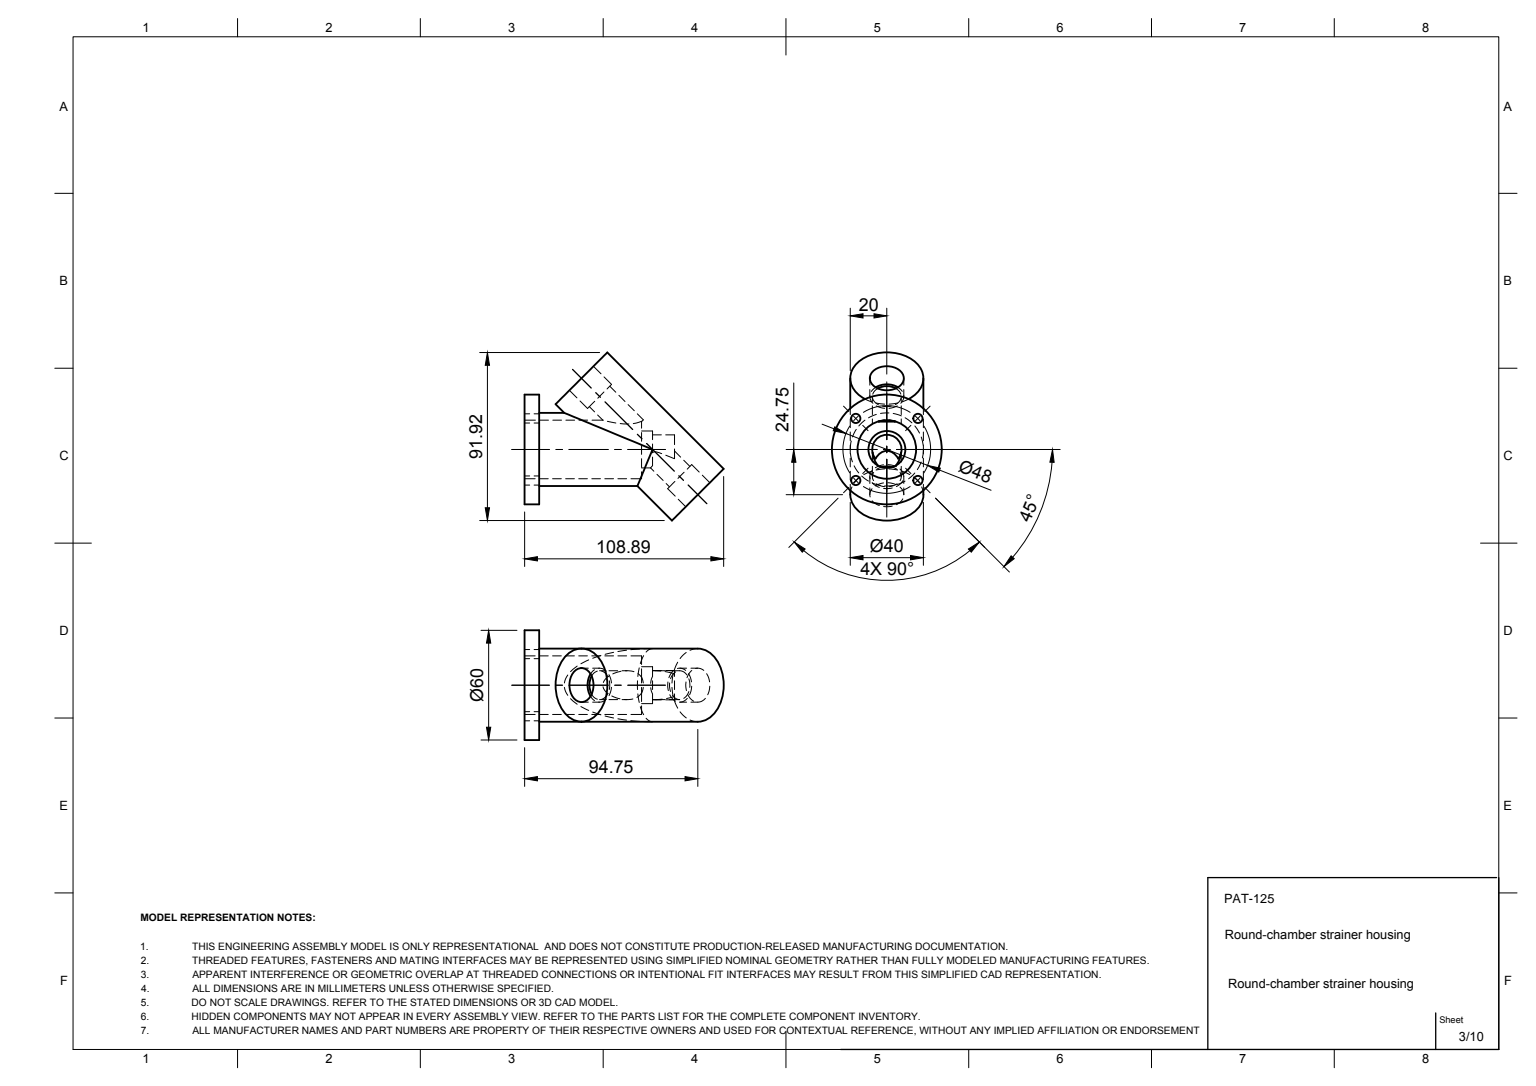
ISO-10303-21;
HEADER;
/* Generated by software containing ST-Developer
 * from STEP Tools, Inc. (www.steptools.com) 
 */

FILE_DESCRIPTION(
/* description */ ('Y-strainer with drain'),
/* implementation_level */ '2;1');

FILE_NAME(
/* name */ 'Round-chamber strainer housing.step',
/* time_stamp */ '2026-10-28T00:41:55-07:00',
/* author */ (''),
/* organization */ (''),
/* preprocessor_version */ 'ST-DEVELOPER v20.2',
/* originating_system */ 'Autodesk Translation Framework v15.17.0.0',
/* authorisation */ '');

FILE_SCHEMA (('AUTOMOTIVE_DESIGN { 1 0 10303 214 3 1 1 }'));
ENDSEC;

DATA;
#10=MECHANICAL_DESIGN_GEOMETRIC_PRESENTATION_REPRESENTATION('',(#93),#8864);
#75=SHAPE_REPRESENTATION_RELATIONSHIP('SRR','None',#8907,#84);
#84=ADVANCED_BREP_SHAPE_REPRESENTATION('',(#102),#8855);
#93=STYLED_ITEM('',(#9012),#102);
#102=MANIFOLD_SOLID_BREP('Body1',#3383);
#110=B_SPLINE_CURVE_WITH_KNOTS('',3,(#4530,#4531,#4532,#4533,#4534,#4535,
#4536,#4537,#4538,#4539,#4540,#4541,#4542,#4543,#4544,#4545,#4546,#4547,
#4548,#4549),.UNSPECIFIED.,.F.,.F.,(4,2,2,2,2,2,2,2,2,4),(-4.14934014091753,
-3.99654801890952,-3.81097439305959,-3.62540076720966,-3.2542535155098,
-2.75110698726675,-2.2479604590237,-1.9375436083893,-1.7823351830721,-1.6271267577549),
 .UNSPECIFIED.);
#111=B_SPLINE_CURVE_WITH_KNOTS('',3,(#4550,#4551,#4552,#4553,#4554,#4555,
#4556,#4557,#4558,#4559,#4560,#4561,#4562,#4563,#4564,#4565,#4566,#4567,
#4568,#4569,#4570),.UNSPECIFIED.,.F.,.F.,(4,2,2,2,2,3,2,2,2,4),(-1.6271267577549,
-1.4719183324377,-1.3167099071205,-1.00629305648611,-0.503146528243052,
0.,0.371147251699857,0.556720877549785,0.742294503399713,0.895086625004965),
 .UNSPECIFIED.);
#112=B_SPLINE_CURVE_WITH_KNOTS('',3,(#4581,#4582,#4583,#4584,#4585,#4586,
#4587,#4588,#4589,#4590),.UNSPECIFIED.,.F.,.F.,(4,2,2,2,4),(1.74412062919654,
1.93171537626907,2.23482107464905,2.53792677302904,2.72552152010157),
 .UNSPECIFIED.);
#113=B_SPLINE_CURVE_WITH_KNOTS('',3,(#4608,#4609,#4610,#4611,#4612,#4613,
#4614,#4615,#4616,#4617,#4618,#4619,#4620,#4621,#4622,#4623,#4624,#4625,
#4626),.UNSPECIFIED.,.F.,.F.,(4,2,2,2,2,3,2,2,4),(-1.08793576529359,-1.02464359039736,
-0.589129183459348,-0.223538305364611,-0.111769152682306,0.,0.0571948520978316,
0.114389704195663,0.138769598257235),.UNSPECIFIED.);
#114=B_SPLINE_CURVE_WITH_KNOTS('',3,(#4628,#4629,#4630,#4631,#4632,#4633,
#4634,#4635,#4636,#4637,#4638,#4639,#4640,#4641,#4642,#4643,#4644,#4645),
 .UNSPECIFIED.,.F.,.F.,(4,2,2,2,2,2,2,2,4),(2.32433792360818,2.34871781766975,
2.40591266976758,2.46310752186541,2.57487667454772,2.68664582723002,3.05223670532476,
3.48775111226277,3.551043287159),.UNSPECIFIED.);
#319=FACE_BOUND('',#677,.T.);
#320=FACE_BOUND('',#687,.T.);
#321=FACE_BOUND('',#690,.T.);
#322=FACE_BOUND('',#693,.T.);
#323=FACE_BOUND('',#694,.T.);
#324=FACE_BOUND('',#695,.T.);
#325=FACE_BOUND('',#696,.T.);
#326=FACE_BOUND('',#697,.T.);
#327=FACE_BOUND('',#701,.T.);
#328=FACE_BOUND('',#702,.T.);
#329=FACE_BOUND('',#703,.T.);
#330=FACE_BOUND('',#704,.T.);
#331=FACE_BOUND('',#705,.T.);
#332=FACE_BOUND('',#707,.T.);
#333=FACE_BOUND('',#709,.T.);
#334=FACE_BOUND('',#711,.T.);
#456=ELLIPSE('',#3509,1.11722871427475,0.79);
#457=ELLIPSE('',#3511,1.11722871427475,0.79);
#458=ELLIPSE('',#3522,1.11722871427475,0.79);
#459=ELLIPSE('',#3524,1.11722871427475,0.79);
#460=ELLIPSE('',#3527,1.11722871427475,0.79);
#461=ELLIPSE('',#3528,1.11722871427475,0.79);
#462=ELLIPSE('',#3548,5.22625185950551,2.);
#463=ELLIPSE('',#3549,2.16478440058479,2.);
#464=ELLIPSE('',#3550,5.22625185950551,2.);
#465=PLANE('',#3508);
#466=PLANE('',#3515);
#467=PLANE('',#3521);
#468=PLANE('',#3529);
#469=PLANE('',#3535);
#470=PLANE('',#3540);
#471=PLANE('',#3542);
#472=PLANE('',#3551);
#473=PLANE('',#3555);
#474=PLANE('',#3556);
#520=FACE_OUTER_BOUND('',#672,.T.);
#521=FACE_OUTER_BOUND('',#673,.T.);
#522=FACE_OUTER_BOUND('',#674,.T.);
#523=FACE_OUTER_BOUND('',#675,.T.);
#524=FACE_OUTER_BOUND('',#676,.T.);
#525=FACE_OUTER_BOUND('',#678,.T.);
#526=FACE_OUTER_BOUND('',#679,.T.);
#527=FACE_OUTER_BOUND('',#680,.T.);
#528=FACE_OUTER_BOUND('',#681,.T.);
#529=FACE_OUTER_BOUND('',#682,.T.);
#530=FACE_OUTER_BOUND('',#683,.T.);
#531=FACE_OUTER_BOUND('',#684,.T.);
#532=FACE_OUTER_BOUND('',#685,.T.);
#533=FACE_OUTER_BOUND('',#686,.T.);
#534=FACE_OUTER_BOUND('',#688,.T.);
#535=FACE_OUTER_BOUND('',#689,.T.);
#536=FACE_OUTER_BOUND('',#691,.T.);
#537=FACE_OUTER_BOUND('',#692,.T.);
#538=FACE_OUTER_BOUND('',#698,.T.);
#539=FACE_OUTER_BOUND('',#699,.T.);
#540=FACE_OUTER_BOUND('',#700,.T.);
#541=FACE_OUTER_BOUND('',#706,.T.);
#542=FACE_OUTER_BOUND('',#708,.T.);
#543=FACE_OUTER_BOUND('',#710,.T.);
#672=EDGE_LOOP('',(#2194,#2195,#2196,#2197));
#673=EDGE_LOOP('',(#2198,#2199,#2200,#2201));
#674=EDGE_LOOP('',(#2202,#2203,#2204,#2205));
#675=EDGE_LOOP('',(#2206,#2207,#2208,#2209));
#676=EDGE_LOOP('',(#2210,#2211,#2212,#2213));
#677=EDGE_LOOP('',(#2214));
#678=EDGE_LOOP('',(#2215,#2216,#2217,#2218,#2219,#2220));
#679=EDGE_LOOP('',(#2221,#2222,#2223));
#680=EDGE_LOOP('',(#2224,#2225,#2226,#2227,#2228,#2229));
#681=EDGE_LOOP('',(#2230,#2231,#2232,#2233,#2234));
#682=EDGE_LOOP('',(#2235,#2236,#2237,#2238,#2239,#2240,#2241,#2242,#2243,
#2244));
#683=EDGE_LOOP('',(#2245,#2246,#2247));
#684=EDGE_LOOP('',(#2248,#2249,#2250,#2251));
#685=EDGE_LOOP('',(#2252,#2253,#2254,#2255));
#686=EDGE_LOOP('',(#2256));
#687=EDGE_LOOP('',(#2257));
#688=EDGE_LOOP('',(#2258,#2259,#2260,#2261));
#689=EDGE_LOOP('',(#2262));
#690=EDGE_LOOP('',(#2263));
#691=EDGE_LOOP('',(#2264,#2265,#2266,#2267,#2268,#2269,#2270,#2271,#2272));
#692=EDGE_LOOP('',(#2273));
#693=EDGE_LOOP('',(#2274));
#694=EDGE_LOOP('',(#2275));
#695=EDGE_LOOP('',(#2276));
#696=EDGE_LOOP('',(#2277));
#697=EDGE_LOOP('',(#2278));
#698=EDGE_LOOP('',(#2279,#2280,#2281,#2282));
#699=EDGE_LOOP('',(#2283,#2284,#2285,#2286,#2287,#2288));
#700=EDGE_LOOP('',(#2289));
#701=EDGE_LOOP('',(#2290));
#702=EDGE_LOOP('',(#2291));
#703=EDGE_LOOP('',(#2292));
#704=EDGE_LOOP('',(#2293));
#705=EDGE_LOOP('',(#2294));
#706=EDGE_LOOP('',(#2295,#2296,#2297,#2298));
#707=EDGE_LOOP('',(#2299,#2300,#2301));
#708=EDGE_LOOP('',(#2302));
#709=EDGE_LOOP('',(#2303));
#710=EDGE_LOOP('',(#2304));
#711=EDGE_LOOP('',(#2305));
#961=LINE('',#4497,#1124);
#962=LINE('',#4503,#1125);
#963=LINE('',#4509,#1126);
#964=LINE('',#4515,#1127);
#965=LINE('',#4525,#1128);
#966=LINE('',#4572,#1129);
#967=LINE('',#4593,#1130);
#968=LINE('',#4605,#1131);
#969=LINE('',#4654,#1132);
#970=LINE('',#4663,#1133);
#971=LINE('',#4667,#1134);
#972=LINE('',#4676,#1135);
#973=LINE('',#4679,#1136);
#974=LINE('',#4690,#1137);
#1124=VECTOR('',#3781,0.25);
#1125=VECTOR('',#3788,0.25);
#1126=VECTOR('',#3795,0.25);
#1127=VECTOR('',#3802,0.25);
#1128=VECTOR('',#3813,1.);
#1129=VECTOR('',#3818,1.6);
#1130=VECTOR('',#3831,1.01);
#1131=VECTOR('',#3846,0.79);
#1132=VECTOR('',#3861,0.93);
#1133=VECTOR('',#3872,0.93);
#1134=VECTOR('',#3879,0.79);
#1135=VECTOR('',#3890,3.);
#1136=VECTOR('',#3893,2.);
#1137=VECTOR('',#3906,2.);
#1287=CIRCLE('',#3497,0.25);
#1288=CIRCLE('',#3498,0.25);
#1289=CIRCLE('',#3500,0.25);
#1290=CIRCLE('',#3501,0.25);
#1291=CIRCLE('',#3503,0.25);
#1292=CIRCLE('',#3504,0.25);
#1293=CIRCLE('',#3506,0.25);
#1294=CIRCLE('',#3507,0.25);
#1295=CIRCLE('',#3510,1.6);
#1296=CIRCLE('',#3512,1.01);
#1297=CIRCLE('',#3514,1.6);
#1298=CIRCLE('',#3516,0.79);
#1299=CIRCLE('',#3517,0.79);
#1300=CIRCLE('',#3519,1.01);
#1301=CIRCLE('',#3520,1.01);
#1302=CIRCLE('',#3523,0.8);
#1303=CIRCLE('',#3526,0.79);
#1304=CIRCLE('',#3530,0.8);
#1305=CIRCLE('',#3533,0.93);
#1306=CIRCLE('',#3534,0.93);
#1307=CIRCLE('',#3536,0.79);
#1308=CIRCLE('',#3538,0.93);
#1309=CIRCLE('',#3539,0.93);
#1310=CIRCLE('',#3543,3.);
#1311=CIRCLE('',#3544,2.);
#1312=CIRCLE('',#3546,3.);
#1313=CIRCLE('',#3553,2.);
#1314=CIRCLE('',#3554,2.);
#1379=VERTEX_POINT('',#4494);
#1380=VERTEX_POINT('',#4496);
#1381=VERTEX_POINT('',#4500);
#1382=VERTEX_POINT('',#4502);
#1383=VERTEX_POINT('',#4506);
#1384=VERTEX_POINT('',#4508);
#1385=VERTEX_POINT('',#4512);
#1386=VERTEX_POINT('',#4514);
#1387=VERTEX_POINT('',#4518);
#1388=VERTEX_POINT('',#4519);
#1389=VERTEX_POINT('',#4521);
#1390=VERTEX_POINT('',#4523);
#1391=VERTEX_POINT('',#4526);
#1392=VERTEX_POINT('',#4529);
#1393=VERTEX_POINT('',#4571);
#1394=VERTEX_POINT('',#4575);
#1395=VERTEX_POINT('',#4579);
#1396=VERTEX_POINT('',#4580);
#1397=VERTEX_POINT('',#4591);
#1398=VERTEX_POINT('',#4596);
#1399=VERTEX_POINT('',#4598);
#1400=VERTEX_POINT('',#4602);
#1401=VERTEX_POINT('',#4604);
#1402=VERTEX_POINT('',#4606);
#1403=VERTEX_POINT('',#4627);
#1404=VERTEX_POINT('',#4651);
#1405=VERTEX_POINT('',#4653);
#1406=VERTEX_POINT('',#4657);
#1407=VERTEX_POINT('',#4660);
#1408=VERTEX_POINT('',#4662);
#1409=VERTEX_POINT('',#4669);
#1410=VERTEX_POINT('',#4671);
#1411=VERTEX_POINT('',#4674);
#1412=VERTEX_POINT('',#4678);
#1413=VERTEX_POINT('',#4680);
#1414=VERTEX_POINT('',#4682);
#1415=VERTEX_POINT('',#4687);
#1416=VERTEX_POINT('',#4689);
#1721=EDGE_CURVE('',#1379,#1379,#1287,.T.);
#1722=EDGE_CURVE('',#1379,#1380,#961,.T.);
#1723=EDGE_CURVE('',#1380,#1380,#1288,.T.);
#1724=EDGE_CURVE('',#1381,#1381,#1289,.T.);
#1725=EDGE_CURVE('',#1381,#1382,#962,.T.);
#1726=EDGE_CURVE('',#1382,#1382,#1290,.T.);
#1727=EDGE_CURVE('',#1383,#1383,#1291,.T.);
#1728=EDGE_CURVE('',#1383,#1384,#963,.T.);
#1729=EDGE_CURVE('',#1384,#1384,#1292,.T.);
#1730=EDGE_CURVE('',#1385,#1385,#1293,.T.);
#1731=EDGE_CURVE('',#1385,#1386,#964,.T.);
#1732=EDGE_CURVE('',#1386,#1386,#1294,.T.);
#1733=EDGE_CURVE('',#1387,#1388,#456,.T.);
#1734=EDGE_CURVE('',#1387,#1389,#1295,.T.);
#1735=EDGE_CURVE('',#1390,#1389,#457,.T.);
#1736=EDGE_CURVE('',#1388,#1390,#965,.T.);
#1737=EDGE_CURVE('',#1391,#1391,#1296,.T.);
#1738=EDGE_CURVE('',#1389,#1392,#110,.T.);
#1739=EDGE_CURVE('',#1392,#1387,#111,.T.);
#1740=EDGE_CURVE('',#1392,#1393,#966,.T.);
#1741=EDGE_CURVE('',#1393,#1393,#1297,.T.);
#1742=EDGE_CURVE('',#1390,#1394,#1298,.T.);
#1743=EDGE_CURVE('',#1394,#1388,#1299,.T.);
#1744=EDGE_CURVE('',#1395,#1396,#112,.T.);
#1745=EDGE_CURVE('',#1397,#1395,#1300,.T.);
#1746=EDGE_CURVE('',#1397,#1391,#967,.T.);
#1747=EDGE_CURVE('',#1396,#1397,#1301,.T.);
#1748=EDGE_CURVE('',#1398,#1395,#458,.T.);
#1749=EDGE_CURVE('',#1399,#1398,#1302,.T.);
#1750=EDGE_CURVE('',#1396,#1399,#459,.T.);
#1751=EDGE_CURVE('',#1400,#1400,#1303,.T.);
#1752=EDGE_CURVE('',#1400,#1401,#968,.T.);
#1753=EDGE_CURVE('',#1401,#1402,#460,.T.);
#1754=EDGE_CURVE('',#1402,#1398,#113,.T.);
#1755=EDGE_CURVE('',#1399,#1403,#114,.T.);
#1756=EDGE_CURVE('',#1403,#1401,#461,.T.);
#1757=EDGE_CURVE('',#1403,#1402,#1304,.T.);
#1758=EDGE_CURVE('',#1404,#1404,#1305,.T.);
#1759=EDGE_CURVE('',#1404,#1405,#969,.T.);
#1760=EDGE_CURVE('',#1405,#1405,#1306,.T.);
#1761=EDGE_CURVE('',#1406,#1406,#1307,.T.);
#1762=EDGE_CURVE('',#1407,#1407,#1308,.T.);
#1763=EDGE_CURVE('',#1407,#1408,#970,.T.);
#1764=EDGE_CURVE('',#1408,#1408,#1309,.T.);
#1765=EDGE_CURVE('',#1394,#1406,#971,.T.);
#1766=EDGE_CURVE('',#1409,#1409,#1310,.T.);
#1767=EDGE_CURVE('',#1410,#1410,#1311,.T.);
#1768=EDGE_CURVE('',#1411,#1411,#1312,.T.);
#1769=EDGE_CURVE('',#1411,#1409,#972,.T.);
#1770=EDGE_CURVE('',#1410,#1412,#973,.T.);
#1771=EDGE_CURVE('',#1413,#1412,#462,.T.);
#1772=EDGE_CURVE('',#1414,#1413,#463,.T.);
#1773=EDGE_CURVE('',#1412,#1414,#464,.T.);
#1774=EDGE_CURVE('',#1415,#1415,#1313,.T.);
#1775=EDGE_CURVE('',#1415,#1416,#974,.T.);
#1776=EDGE_CURVE('',#1416,#1416,#1314,.T.);
#2194=ORIENTED_EDGE('',*,*,#1721,.F.);
#2195=ORIENTED_EDGE('',*,*,#1722,.T.);
#2196=ORIENTED_EDGE('',*,*,#1723,.F.);
#2197=ORIENTED_EDGE('',*,*,#1722,.F.);
#2198=ORIENTED_EDGE('',*,*,#1724,.F.);
#2199=ORIENTED_EDGE('',*,*,#1725,.T.);
#2200=ORIENTED_EDGE('',*,*,#1726,.F.);
#2201=ORIENTED_EDGE('',*,*,#1725,.F.);
#2202=ORIENTED_EDGE('',*,*,#1727,.F.);
#2203=ORIENTED_EDGE('',*,*,#1728,.T.);
#2204=ORIENTED_EDGE('',*,*,#1729,.F.);
#2205=ORIENTED_EDGE('',*,*,#1728,.F.);
#2206=ORIENTED_EDGE('',*,*,#1730,.F.);
#2207=ORIENTED_EDGE('',*,*,#1731,.T.);
#2208=ORIENTED_EDGE('',*,*,#1732,.F.);
#2209=ORIENTED_EDGE('',*,*,#1731,.F.);
#2210=ORIENTED_EDGE('',*,*,#1733,.F.);
#2211=ORIENTED_EDGE('',*,*,#1734,.T.);
#2212=ORIENTED_EDGE('',*,*,#1735,.F.);
#2213=ORIENTED_EDGE('',*,*,#1736,.F.);
#2214=ORIENTED_EDGE('',*,*,#1737,.F.);
#2215=ORIENTED_EDGE('',*,*,#1738,.F.);
#2216=ORIENTED_EDGE('',*,*,#1734,.F.);
#2217=ORIENTED_EDGE('',*,*,#1739,.F.);
#2218=ORIENTED_EDGE('',*,*,#1740,.T.);
#2219=ORIENTED_EDGE('',*,*,#1741,.F.);
#2220=ORIENTED_EDGE('',*,*,#1740,.F.);
#2221=ORIENTED_EDGE('',*,*,#1736,.T.);
#2222=ORIENTED_EDGE('',*,*,#1742,.T.);
#2223=ORIENTED_EDGE('',*,*,#1743,.T.);
#2224=ORIENTED_EDGE('',*,*,#1744,.F.);
#2225=ORIENTED_EDGE('',*,*,#1745,.F.);
#2226=ORIENTED_EDGE('',*,*,#1746,.T.);
#2227=ORIENTED_EDGE('',*,*,#1737,.T.);
#2228=ORIENTED_EDGE('',*,*,#1746,.F.);
#2229=ORIENTED_EDGE('',*,*,#1747,.F.);
#2230=ORIENTED_EDGE('',*,*,#1748,.F.);
#2231=ORIENTED_EDGE('',*,*,#1749,.F.);
#2232=ORIENTED_EDGE('',*,*,#1750,.F.);
#2233=ORIENTED_EDGE('',*,*,#1747,.T.);
#2234=ORIENTED_EDGE('',*,*,#1745,.T.);
#2235=ORIENTED_EDGE('',*,*,#1751,.T.);
#2236=ORIENTED_EDGE('',*,*,#1752,.T.);
#2237=ORIENTED_EDGE('',*,*,#1753,.T.);
#2238=ORIENTED_EDGE('',*,*,#1754,.T.);
#2239=ORIENTED_EDGE('',*,*,#1748,.T.);
#2240=ORIENTED_EDGE('',*,*,#1744,.T.);
#2241=ORIENTED_EDGE('',*,*,#1750,.T.);
#2242=ORIENTED_EDGE('',*,*,#1755,.T.);
#2243=ORIENTED_EDGE('',*,*,#1756,.T.);
#2244=ORIENTED_EDGE('',*,*,#1752,.F.);
#2245=ORIENTED_EDGE('',*,*,#1756,.F.);
#2246=ORIENTED_EDGE('',*,*,#1757,.T.);
#2247=ORIENTED_EDGE('',*,*,#1753,.F.);
#2248=ORIENTED_EDGE('',*,*,#1755,.F.);
#2249=ORIENTED_EDGE('',*,*,#1749,.T.);
#2250=ORIENTED_EDGE('',*,*,#1754,.F.);
#2251=ORIENTED_EDGE('',*,*,#1757,.F.);
#2252=ORIENTED_EDGE('',*,*,#1758,.F.);
#2253=ORIENTED_EDGE('',*,*,#1759,.T.);
#2254=ORIENTED_EDGE('',*,*,#1760,.F.);
#2255=ORIENTED_EDGE('',*,*,#1759,.F.);
#2256=ORIENTED_EDGE('',*,*,#1758,.T.);
#2257=ORIENTED_EDGE('',*,*,#1761,.F.);
#2258=ORIENTED_EDGE('',*,*,#1762,.F.);
#2259=ORIENTED_EDGE('',*,*,#1763,.T.);
#2260=ORIENTED_EDGE('',*,*,#1764,.T.);
#2261=ORIENTED_EDGE('',*,*,#1763,.F.);
#2262=ORIENTED_EDGE('',*,*,#1764,.F.);
#2263=ORIENTED_EDGE('',*,*,#1751,.F.);
#2264=ORIENTED_EDGE('',*,*,#1733,.T.);
#2265=ORIENTED_EDGE('',*,*,#1743,.F.);
#2266=ORIENTED_EDGE('',*,*,#1765,.T.);
#2267=ORIENTED_EDGE('',*,*,#1761,.T.);
#2268=ORIENTED_EDGE('',*,*,#1765,.F.);
#2269=ORIENTED_EDGE('',*,*,#1742,.F.);
#2270=ORIENTED_EDGE('',*,*,#1735,.T.);
#2271=ORIENTED_EDGE('',*,*,#1738,.T.);
#2272=ORIENTED_EDGE('',*,*,#1739,.T.);
#2273=ORIENTED_EDGE('',*,*,#1766,.F.);
#2274=ORIENTED_EDGE('',*,*,#1721,.T.);
#2275=ORIENTED_EDGE('',*,*,#1724,.T.);
#2276=ORIENTED_EDGE('',*,*,#1727,.T.);
#2277=ORIENTED_EDGE('',*,*,#1730,.T.);
#2278=ORIENTED_EDGE('',*,*,#1767,.F.);
#2279=ORIENTED_EDGE('',*,*,#1768,.F.);
#2280=ORIENTED_EDGE('',*,*,#1769,.T.);
#2281=ORIENTED_EDGE('',*,*,#1766,.T.);
#2282=ORIENTED_EDGE('',*,*,#1769,.F.);
#2283=ORIENTED_EDGE('',*,*,#1767,.T.);
#2284=ORIENTED_EDGE('',*,*,#1770,.T.);
#2285=ORIENTED_EDGE('',*,*,#1771,.F.);
#2286=ORIENTED_EDGE('',*,*,#1772,.F.);
#2287=ORIENTED_EDGE('',*,*,#1773,.F.);
#2288=ORIENTED_EDGE('',*,*,#1770,.F.);
#2289=ORIENTED_EDGE('',*,*,#1768,.T.);
#2290=ORIENTED_EDGE('',*,*,#1723,.T.);
#2291=ORIENTED_EDGE('',*,*,#1726,.T.);
#2292=ORIENTED_EDGE('',*,*,#1729,.T.);
#2293=ORIENTED_EDGE('',*,*,#1732,.T.);
#2294=ORIENTED_EDGE('',*,*,#1741,.T.);
#2295=ORIENTED_EDGE('',*,*,#1774,.F.);
#2296=ORIENTED_EDGE('',*,*,#1775,.T.);
#2297=ORIENTED_EDGE('',*,*,#1776,.T.);
#2298=ORIENTED_EDGE('',*,*,#1775,.F.);
#2299=ORIENTED_EDGE('',*,*,#1771,.T.);
#2300=ORIENTED_EDGE('',*,*,#1773,.T.);
#2301=ORIENTED_EDGE('',*,*,#1772,.T.);
#2302=ORIENTED_EDGE('',*,*,#1774,.T.);
#2303=ORIENTED_EDGE('',*,*,#1760,.T.);
#2304=ORIENTED_EDGE('',*,*,#1776,.F.);
#2305=ORIENTED_EDGE('',*,*,#1762,.T.);
#3140=CYLINDRICAL_SURFACE('',#3496,0.25);
#3141=CYLINDRICAL_SURFACE('',#3499,0.25);
#3142=CYLINDRICAL_SURFACE('',#3502,0.25);
#3143=CYLINDRICAL_SURFACE('',#3505,0.25);
#3144=CYLINDRICAL_SURFACE('',#3513,1.6);
#3145=CYLINDRICAL_SURFACE('',#3518,1.01);
#3146=CYLINDRICAL_SURFACE('',#3525,0.79);
#3147=CYLINDRICAL_SURFACE('',#3531,0.8);
#3148=CYLINDRICAL_SURFACE('',#3532,0.93);
#3149=CYLINDRICAL_SURFACE('',#3537,0.93);
#3150=CYLINDRICAL_SURFACE('',#3541,0.79);
#3151=CYLINDRICAL_SURFACE('',#3545,3.);
#3152=CYLINDRICAL_SURFACE('',#3547,2.);
#3153=CYLINDRICAL_SURFACE('',#3552,2.);
#3231=ADVANCED_FACE('',(#520),#3140,.F.);
#3232=ADVANCED_FACE('',(#521),#3141,.F.);
#3233=ADVANCED_FACE('',(#522),#3142,.F.);
#3234=ADVANCED_FACE('',(#523),#3143,.F.);
#3235=ADVANCED_FACE('',(#524,#319),#465,.T.);
#3236=ADVANCED_FACE('',(#525),#3144,.F.);
#3237=ADVANCED_FACE('',(#526),#466,.T.);
#3238=ADVANCED_FACE('',(#527),#3145,.F.);
#3239=ADVANCED_FACE('',(#528),#467,.T.);
#3240=ADVANCED_FACE('',(#529),#3146,.F.);
#3241=ADVANCED_FACE('',(#530),#468,.T.);
#3242=ADVANCED_FACE('',(#531),#3147,.F.);
#3243=ADVANCED_FACE('',(#532),#3148,.F.);
#3244=ADVANCED_FACE('',(#533,#320),#469,.T.);
#3245=ADVANCED_FACE('',(#534),#3149,.F.);
#3246=ADVANCED_FACE('',(#535,#321),#470,.F.);
#3247=ADVANCED_FACE('',(#536),#3150,.F.);
#3248=ADVANCED_FACE('',(#537,#322,#323,#324,#325,#326),#471,.F.);
#3249=ADVANCED_FACE('',(#538),#3151,.T.);
#3250=ADVANCED_FACE('',(#539),#3152,.T.);
#3251=ADVANCED_FACE('',(#540,#327,#328,#329,#330,#331),#472,.T.);
#3252=ADVANCED_FACE('',(#541,#332),#3153,.T.);
#3253=ADVANCED_FACE('',(#542,#333),#473,.T.);
#3254=ADVANCED_FACE('',(#543,#334),#474,.F.);
#3383=CLOSED_SHELL('',(#3231,#3232,#3233,#3234,#3235,#3236,#3237,#3238,
#3239,#3240,#3241,#3242,#3243,#3244,#3245,#3246,#3247,#3248,#3249,#3250,
#3251,#3252,#3253,#3254));
#3495=AXIS2_PLACEMENT_3D('',#4492,#3775,#3776);
#3496=AXIS2_PLACEMENT_3D('',#4493,#3777,#3778);
#3497=AXIS2_PLACEMENT_3D('',#4495,#3779,#3780);
#3498=AXIS2_PLACEMENT_3D('',#4498,#3782,#3783);
#3499=AXIS2_PLACEMENT_3D('',#4499,#3784,#3785);
#3500=AXIS2_PLACEMENT_3D('',#4501,#3786,#3787);
#3501=AXIS2_PLACEMENT_3D('',#4504,#3789,#3790);
#3502=AXIS2_PLACEMENT_3D('',#4505,#3791,#3792);
#3503=AXIS2_PLACEMENT_3D('',#4507,#3793,#3794);
#3504=AXIS2_PLACEMENT_3D('',#4510,#3796,#3797);
#3505=AXIS2_PLACEMENT_3D('',#4511,#3798,#3799);
#3506=AXIS2_PLACEMENT_3D('',#4513,#3800,#3801);
#3507=AXIS2_PLACEMENT_3D('',#4516,#3803,#3804);
#3508=AXIS2_PLACEMENT_3D('',#4517,#3805,#3806);
#3509=AXIS2_PLACEMENT_3D('',#4520,#3807,#3808);
#3510=AXIS2_PLACEMENT_3D('',#4522,#3809,#3810);
#3511=AXIS2_PLACEMENT_3D('',#4524,#3811,#3812);
#3512=AXIS2_PLACEMENT_3D('',#4527,#3814,#3815);
#3513=AXIS2_PLACEMENT_3D('',#4528,#3816,#3817);
#3514=AXIS2_PLACEMENT_3D('',#4573,#3819,#3820);
#3515=AXIS2_PLACEMENT_3D('',#4574,#3821,#3822);
#3516=AXIS2_PLACEMENT_3D('',#4576,#3823,#3824);
#3517=AXIS2_PLACEMENT_3D('',#4577,#3825,#3826);
#3518=AXIS2_PLACEMENT_3D('',#4578,#3827,#3828);
#3519=AXIS2_PLACEMENT_3D('',#4592,#3829,#3830);
#3520=AXIS2_PLACEMENT_3D('',#4594,#3832,#3833);
#3521=AXIS2_PLACEMENT_3D('',#4595,#3834,#3835);
#3522=AXIS2_PLACEMENT_3D('',#4597,#3836,#3837);
#3523=AXIS2_PLACEMENT_3D('',#4599,#3838,#3839);
#3524=AXIS2_PLACEMENT_3D('',#4600,#3840,#3841);
#3525=AXIS2_PLACEMENT_3D('',#4601,#3842,#3843);
#3526=AXIS2_PLACEMENT_3D('',#4603,#3844,#3845);
#3527=AXIS2_PLACEMENT_3D('',#4607,#3847,#3848);
#3528=AXIS2_PLACEMENT_3D('',#4646,#3849,#3850);
#3529=AXIS2_PLACEMENT_3D('',#4647,#3851,#3852);
#3530=AXIS2_PLACEMENT_3D('',#4648,#3853,#3854);
#3531=AXIS2_PLACEMENT_3D('',#4649,#3855,#3856);
#3532=AXIS2_PLACEMENT_3D('',#4650,#3857,#3858);
#3533=AXIS2_PLACEMENT_3D('',#4652,#3859,#3860);
#3534=AXIS2_PLACEMENT_3D('',#4655,#3862,#3863);
#3535=AXIS2_PLACEMENT_3D('',#4656,#3864,#3865);
#3536=AXIS2_PLACEMENT_3D('',#4658,#3866,#3867);
#3537=AXIS2_PLACEMENT_3D('',#4659,#3868,#3869);
#3538=AXIS2_PLACEMENT_3D('',#4661,#3870,#3871);
#3539=AXIS2_PLACEMENT_3D('',#4664,#3873,#3874);
#3540=AXIS2_PLACEMENT_3D('',#4665,#3875,#3876);
#3541=AXIS2_PLACEMENT_3D('',#4666,#3877,#3878);
#3542=AXIS2_PLACEMENT_3D('',#4668,#3880,#3881);
#3543=AXIS2_PLACEMENT_3D('',#4670,#3882,#3883);
#3544=AXIS2_PLACEMENT_3D('',#4672,#3884,#3885);
#3545=AXIS2_PLACEMENT_3D('',#4673,#3886,#3887);
#3546=AXIS2_PLACEMENT_3D('',#4675,#3888,#3889);
#3547=AXIS2_PLACEMENT_3D('',#4677,#3891,#3892);
#3548=AXIS2_PLACEMENT_3D('',#4681,#3894,#3895);
#3549=AXIS2_PLACEMENT_3D('',#4683,#3896,#3897);
#3550=AXIS2_PLACEMENT_3D('',#4684,#3898,#3899);
#3551=AXIS2_PLACEMENT_3D('',#4685,#3900,#3901);
#3552=AXIS2_PLACEMENT_3D('',#4686,#3902,#3903);
#3553=AXIS2_PLACEMENT_3D('',#4688,#3904,#3905);
#3554=AXIS2_PLACEMENT_3D('',#4691,#3907,#3908);
#3555=AXIS2_PLACEMENT_3D('',#4692,#3909,#3910);
#3556=AXIS2_PLACEMENT_3D('',#4693,#3911,#3912);
#3775=DIRECTION('axis',(0.,0.,1.));
#3776=DIRECTION('refdir',(1.,0.,0.));
#3777=DIRECTION('center_axis',(0.707106781186548,0.,-0.707106781186547));
#3778=DIRECTION('ref_axis',(-0.707106781186547,0.,-0.707106781186548));
#3779=DIRECTION('center_axis',(0.707106781186548,0.,-0.707106781186547));
#3780=DIRECTION('ref_axis',(-0.707106781186547,0.,-0.707106781186548));
#3781=DIRECTION('',(0.707106781186548,0.,-0.707106781186547));
#3782=DIRECTION('center_axis',(-0.707106781186548,0.,0.707106781186547));
#3783=DIRECTION('ref_axis',(-0.707106781186547,0.,-0.707106781186548));
#3784=DIRECTION('center_axis',(0.707106781186548,0.,-0.707106781186547));
#3785=DIRECTION('ref_axis',(-0.707106781186547,0.,-0.707106781186548));
#3786=DIRECTION('center_axis',(0.707106781186548,0.,-0.707106781186547));
#3787=DIRECTION('ref_axis',(-0.707106781186547,0.,-0.707106781186548));
#3788=DIRECTION('',(0.707106781186548,0.,-0.707106781186547));
#3789=DIRECTION('center_axis',(-0.707106781186548,0.,0.707106781186547));
#3790=DIRECTION('ref_axis',(-0.707106781186547,0.,-0.707106781186548));
#3791=DIRECTION('center_axis',(0.707106781186548,0.,-0.707106781186547));
#3792=DIRECTION('ref_axis',(-0.707106781186547,0.,-0.707106781186548));
#3793=DIRECTION('center_axis',(0.707106781186548,0.,-0.707106781186547));
#3794=DIRECTION('ref_axis',(-0.707106781186547,0.,-0.707106781186548));
#3795=DIRECTION('',(0.707106781186548,0.,-0.707106781186547));
#3796=DIRECTION('center_axis',(-0.707106781186548,0.,0.707106781186547));
#3797=DIRECTION('ref_axis',(-0.707106781186547,0.,-0.707106781186548));
#3798=DIRECTION('center_axis',(0.707106781186548,0.,-0.707106781186547));
#3799=DIRECTION('ref_axis',(-0.707106781186547,0.,-0.707106781186548));
#3800=DIRECTION('center_axis',(0.707106781186548,0.,-0.707106781186547));
#3801=DIRECTION('ref_axis',(-0.707106781186547,0.,-0.707106781186548));
#3802=DIRECTION('',(0.707106781186548,0.,-0.707106781186547));
#3803=DIRECTION('center_axis',(-0.707106781186548,0.,0.707106781186547));
#3804=DIRECTION('ref_axis',(-0.707106781186547,0.,-0.707106781186548));
#3805=DIRECTION('center_axis',(0.707106781186548,0.,-0.707106781186547));
#3806=DIRECTION('ref_axis',(-0.707106781186547,0.,-0.707106781186548));
#3807=DIRECTION('center_axis',(0.707106781186548,0.,-0.707106781186547));
#3808=DIRECTION('ref_axis',(-0.707106781186547,0.,-0.707106781186548));
#3809=DIRECTION('center_axis',(0.707106781186548,0.,-0.707106781186547));
#3810=DIRECTION('ref_axis',(-0.707106781186547,0.,-0.707106781186548));
#3811=DIRECTION('center_axis',(0.707106781186548,0.,-0.707106781186547));
#3812=DIRECTION('ref_axis',(-0.707106781186547,0.,-0.707106781186548));
#3813=DIRECTION('',(0.,1.,0.));
#3814=DIRECTION('center_axis',(0.707106781186548,0.,-0.707106781186547));
#3815=DIRECTION('ref_axis',(-0.707106781186547,0.,-0.707106781186548));
#3816=DIRECTION('center_axis',(0.707106781186548,0.,-0.707106781186547));
#3817=DIRECTION('ref_axis',(-0.707106781186547,0.,-0.707106781186548));
#3818=DIRECTION('',(0.707106781186548,0.,-0.707106781186547));
#3819=DIRECTION('center_axis',(-0.707106781186548,0.,0.707106781186547));
#3820=DIRECTION('ref_axis',(-0.707106781186547,0.,-0.707106781186548));
#3821=DIRECTION('center_axis',(1.,0.,0.));
#3822=DIRECTION('ref_axis',(0.,0.,-1.));
#3823=DIRECTION('center_axis',(1.,0.,0.));
#3824=DIRECTION('ref_axis',(0.,0.,-1.));
#3825=DIRECTION('center_axis',(1.,0.,0.));
#3826=DIRECTION('ref_axis',(0.,0.,-1.));
#3827=DIRECTION('center_axis',(0.707106781186548,0.,-0.707106781186547));
#3828=DIRECTION('ref_axis',(-0.707106781186547,0.,-0.707106781186548));
#3829=DIRECTION('center_axis',(0.707106781186548,0.,-0.707106781186547));
#3830=DIRECTION('ref_axis',(-0.707106781186547,0.,-0.707106781186548));
#3831=DIRECTION('',(0.707106781186548,0.,-0.707106781186547));
#3832=DIRECTION('center_axis',(0.707106781186548,0.,-0.707106781186547));
#3833=DIRECTION('ref_axis',(-0.707106781186547,0.,-0.707106781186548));
#3834=DIRECTION('center_axis',(0.707106781186548,0.,-0.707106781186547));
#3835=DIRECTION('ref_axis',(-0.707106781186547,0.,-0.707106781186548));
#3836=DIRECTION('center_axis',(0.707106781186548,0.,-0.707106781186547));
#3837=DIRECTION('ref_axis',(-0.707106781186547,0.,-0.707106781186548));
#3838=DIRECTION('center_axis',(0.707106781186548,0.,-0.707106781186547));
#3839=DIRECTION('ref_axis',(-0.707106781186547,0.,-0.707106781186548));
#3840=DIRECTION('center_axis',(0.707106781186548,0.,-0.707106781186547));
#3841=DIRECTION('ref_axis',(-0.707106781186547,0.,-0.707106781186548));
#3842=DIRECTION('center_axis',(1.,0.,0.));
#3843=DIRECTION('ref_axis',(0.,0.,-1.));
#3844=DIRECTION('center_axis',(-1.,0.,0.));
#3845=DIRECTION('ref_axis',(0.,0.,-1.));
#3846=DIRECTION('',(1.,0.,0.));
#3847=DIRECTION('center_axis',(0.707106781186548,0.,-0.707106781186547));
#3848=DIRECTION('ref_axis',(-0.707106781186547,0.,-0.707106781186548));
#3849=DIRECTION('center_axis',(0.707106781186548,0.,-0.707106781186547));
#3850=DIRECTION('ref_axis',(-0.707106781186547,0.,-0.707106781186548));
#3851=DIRECTION('center_axis',(0.707106781186548,0.,-0.707106781186547));
#3852=DIRECTION('ref_axis',(-0.707106781186547,0.,-0.707106781186548));
#3853=DIRECTION('center_axis',(0.707106781186548,0.,-0.707106781186547));
#3854=DIRECTION('ref_axis',(-0.707106781186547,0.,-0.707106781186548));
#3855=DIRECTION('center_axis',(0.707106781186548,0.,-0.707106781186547));
#3856=DIRECTION('ref_axis',(0.707106781186547,5.66553889764798E-16,0.707106781186548));
#3857=DIRECTION('center_axis',(1.,0.,0.));
#3858=DIRECTION('ref_axis',(0.,0.,-1.));
#3859=DIRECTION('center_axis',(1.,0.,0.));
#3860=DIRECTION('ref_axis',(0.,0.,-1.));
#3861=DIRECTION('',(1.,0.,0.));
#3862=DIRECTION('center_axis',(-1.,0.,0.));
#3863=DIRECTION('ref_axis',(0.,0.,-1.));
#3864=DIRECTION('center_axis',(1.,0.,0.));
#3865=DIRECTION('ref_axis',(0.,0.,-1.));
#3866=DIRECTION('center_axis',(1.,0.,0.));
#3867=DIRECTION('ref_axis',(0.,0.,-1.));
#3868=DIRECTION('center_axis',(1.,0.,0.));
#3869=DIRECTION('ref_axis',(0.,0.,-1.));
#3870=DIRECTION('center_axis',(1.,0.,0.));
#3871=DIRECTION('ref_axis',(0.,0.,-1.));
#3872=DIRECTION('',(1.,0.,0.));
#3873=DIRECTION('center_axis',(1.,0.,0.));
#3874=DIRECTION('ref_axis',(0.,0.,-1.));
#3875=DIRECTION('center_axis',(1.,0.,0.));
#3876=DIRECTION('ref_axis',(0.,0.,-1.));
#3877=DIRECTION('center_axis',(1.,0.,0.));
#3878=DIRECTION('ref_axis',(0.,0.,-1.));
#3879=DIRECTION('',(1.,0.,0.));
#3880=DIRECTION('center_axis',(0.707106781186548,0.,-0.707106781186547));
#3881=DIRECTION('ref_axis',(-0.707106781186547,0.,-0.707106781186548));
#3882=DIRECTION('center_axis',(0.707106781186548,0.,-0.707106781186547));
#3883=DIRECTION('ref_axis',(-0.707106781186547,0.,-0.707106781186548));
#3884=DIRECTION('center_axis',(-0.707106781186548,0.,0.707106781186547));
#3885=DIRECTION('ref_axis',(-0.707106781186547,0.,-0.707106781186548));
#3886=DIRECTION('center_axis',(0.707106781186548,0.,-0.707106781186547));
#3887=DIRECTION('ref_axis',(-0.707106781186547,0.,-0.707106781186548));
#3888=DIRECTION('center_axis',(0.707106781186548,0.,-0.707106781186547));
#3889=DIRECTION('ref_axis',(-0.707106781186547,0.,-0.707106781186548));
#3890=DIRECTION('',(-0.707106781186548,0.,0.707106781186547));
#3891=DIRECTION('center_axis',(0.707106781186548,0.,-0.707106781186547));
#3892=DIRECTION('ref_axis',(-0.707106781186547,0.,-0.707106781186548));
#3893=DIRECTION('',(-0.707106781186548,0.,0.707106781186547));
#3894=DIRECTION('center_axis',(0.38268343236509,0.,0.923879532511287));
#3895=DIRECTION('ref_axis',(-0.923879532511287,0.,0.38268343236509));
#3896=DIRECTION('center_axis',(-0.923879532511287,0.,0.38268343236509));
#3897=DIRECTION('ref_axis',(-0.38268343236509,0.,-0.923879532511287));
#3898=DIRECTION('center_axis',(0.38268343236509,0.,0.923879532511287));
#3899=DIRECTION('ref_axis',(-0.923879532511287,0.,0.38268343236509));
#3900=DIRECTION('center_axis',(0.707106781186548,0.,-0.707106781186547));
#3901=DIRECTION('ref_axis',(-0.707106781186547,0.,-0.707106781186548));
#3902=DIRECTION('center_axis',(1.,0.,0.));
#3903=DIRECTION('ref_axis',(0.,0.,-1.));
#3904=DIRECTION('center_axis',(1.,0.,0.));
#3905=DIRECTION('ref_axis',(0.,0.,-1.));
#3906=DIRECTION('',(-1.,0.,0.));
#3907=DIRECTION('center_axis',(1.,0.,0.));
#3908=DIRECTION('ref_axis',(0.,0.,-1.));
#3909=DIRECTION('center_axis',(1.,0.,0.));
#3910=DIRECTION('ref_axis',(0.,0.,-1.));
#3911=DIRECTION('center_axis',(1.,0.,0.));
#3912=DIRECTION('ref_axis',(0.,0.,-1.));
#4492=CARTESIAN_POINT('',(0.,0.,0.));
#4493=CARTESIAN_POINT('Origin',(2.11335136523794,-1.69705627484771,1.48664863476206));
#4494=CARTESIAN_POINT('',(2.36083873865323,-1.69705627484771,1.59271465194004));
#4495=CARTESIAN_POINT('Origin',(2.1840620433566,-1.69705627484771,1.41593795664341));
#4496=CARTESIAN_POINT('',(2.92652416360247,-1.69705627484771,1.0270292269908));
#4497=CARTESIAN_POINT('',(2.29012806053458,-1.69705627484771,1.6634253300587));
#4498=CARTESIAN_POINT('Origin',(2.74974746830583,-1.69705627484771,0.850252531694168));
#4499=CARTESIAN_POINT('Origin',(2.11335136523794,1.69705627484771,1.48664863476206));
#4500=CARTESIAN_POINT('',(2.36083873865323,1.69705627484771,1.59271465194004));
#4501=CARTESIAN_POINT('Origin',(2.1840620433566,1.69705627484771,1.41593795664341));
#4502=CARTESIAN_POINT('',(2.92652416360247,1.69705627484771,1.0270292269908));
#4503=CARTESIAN_POINT('',(2.29012806053458,1.69705627484771,1.6634253300587));
#4504=CARTESIAN_POINT('Origin',(2.74974746830583,1.69705627484771,0.850252531694167));
#4505=CARTESIAN_POINT('Origin',(4.51335136523794,1.69705627484771,3.88664863476206));
#4506=CARTESIAN_POINT('',(4.76083873865323,1.69705627484771,3.99271465194004));
#4507=CARTESIAN_POINT('Origin',(4.5840620433566,1.69705627484771,3.81593795664341));
#4508=CARTESIAN_POINT('',(5.32652416360247,1.69705627484771,3.42702922699081));
#4509=CARTESIAN_POINT('',(4.69012806053458,1.69705627484771,4.0634253300587));
#4510=CARTESIAN_POINT('Origin',(5.14974746830583,1.69705627484771,3.25025253169417));
#4511=CARTESIAN_POINT('Origin',(4.51335136523794,-1.69705627484771,3.88664863476206));
#4512=CARTESIAN_POINT('',(4.76083873865323,-1.69705627484771,3.99271465194004));
#4513=CARTESIAN_POINT('Origin',(4.5840620433566,-1.69705627484771,3.81593795664341));
#4514=CARTESIAN_POINT('',(5.32652416360247,-1.69705627484771,3.42702922699081));
#4515=CARTESIAN_POINT('',(4.69012806053458,-1.69705627484771,4.0634253300587));
#4516=CARTESIAN_POINT('Origin',(5.14974746830583,-1.69705627484771,3.25025253169417));
#4517=CARTESIAN_POINT('Origin',(-0.575735931288071,0.,6.57573593128807));
#4518=CARTESIAN_POINT('',(0.515222755900927,-0.42381397534026,7.66669461847707));
#4519=CARTESIAN_POINT('',(0.5,-0.446860618394116,7.65147186257614));
#4520=CARTESIAN_POINT('Origin',(-0.151471862576143,0.,7.));
#4521=CARTESIAN_POINT('',(0.515222755900927,0.42381397534026,7.66669461847707));
#4522=CARTESIAN_POINT('Origin',(-0.575735931288071,0.,6.57573593128807));
#4523=CARTESIAN_POINT('',(0.5,0.446860618394116,7.65147186257614));
#4524=CARTESIAN_POINT('Origin',(-0.151471862576143,0.,7.));
#4525=CARTESIAN_POINT('',(0.5,0.,7.65147186257614));
#4526=CARTESIAN_POINT('',(0.138441917710342,-1.23689326713883E-16,7.28991378028648));
#4527=CARTESIAN_POINT('Origin',(-0.575735931288071,0.,6.57573593128807));
#4528=CARTESIAN_POINT('Origin',(-0.575735931288071,0.,6.57573593128807));
#4529=CARTESIAN_POINT('',(2.05274169979695,-7.76612318099432E-18,6.21));
#4530=CARTESIAN_POINT('Ctrl Pts',(0.515222755900927,0.423813975340259,7.66669461847707));
#4531=CARTESIAN_POINT('Ctrl Pts',(0.526116666884646,0.467880373133453,7.63868186014655));
#4532=CARTESIAN_POINT('Ctrl Pts',(0.53939367180672,0.508081707628242,7.60688542097163));
#4533=CARTESIAN_POINT('Ctrl Pts',(0.573486312745389,0.586129881875093,7.53294329022174));
#4534=CARTESIAN_POINT('Ctrl Pts',(0.596451435323986,0.624301170571409,7.48753051107401));
#4535=CARTESIAN_POINT('Ctrl Pts',(0.65156518194746,0.68858835699378,7.39151504429253));
#4536=CARTESIAN_POINT('Ctrl Pts',(0.683747388356032,0.714719578864005,7.34094189934536));
#4537=CARTESIAN_POINT('Ctrl Pts',(0.791807275601753,0.774755581890673,7.18899251283438));
#4538=CARTESIAN_POINT('Ctrl Pts',(0.88020875365155,0.79,7.08748024616524));
#4539=CARTESIAN_POINT('Ctrl Pts',(1.08628177383383,0.79,6.88140722598296));
#4540=CARTESIAN_POINT('Ctrl Pts',(1.22448970987637,0.76321488961253,6.76575702265008));
#4541=CARTESIAN_POINT('Ctrl Pts',(1.5022165321408,0.66455929680406,6.55758880230742));
#4542=CARTESIAN_POINT('Ctrl Pts',(1.64147614223073,0.592948544581024,6.46460220651928));
#4543=CARTESIAN_POINT('Ctrl Pts',(1.83272612115297,0.444293338230863,6.34266823160953));
#4544=CARTESIAN_POINT('Ctrl Pts',(1.90715208192005,0.371863087636435,6.29702949928263));
#4545=CARTESIAN_POINT('Ctrl Pts',(1.98979747291659,0.244143424893146,6.24728394566456));
#4546=CARTESIAN_POINT('Ctrl Pts',(2.01256955325863,0.198394270739821,6.23374920803759));
#4547=CARTESIAN_POINT('Ctrl Pts',(2.04404821289531,0.102192836977527,6.21510689448735));
#4548=CARTESIAN_POINT('Ctrl Pts',(2.05274169979695,0.0517361417724,6.21));
#4549=CARTESIAN_POINT('Ctrl Pts',(2.05274169979695,2.63677968348475E-16,
6.21));
#4550=CARTESIAN_POINT('Ctrl Pts',(2.05274169979695,1.80411241501588E-16,
6.21));
#4551=CARTESIAN_POINT('Ctrl Pts',(2.05274169979695,-0.0517361417723996,
6.21));
#4552=CARTESIAN_POINT('Ctrl Pts',(2.04404821289531,-0.102192836977527,6.21510689448735));
#4553=CARTESIAN_POINT('Ctrl Pts',(2.01256955325863,-0.19839427073982,6.23374920803759));
#4554=CARTESIAN_POINT('Ctrl Pts',(1.98979747291659,-0.244143424893145,6.24728394566456));
#4555=CARTESIAN_POINT('Ctrl Pts',(1.90715208192005,-0.371863087636433,6.29702949928263));
#4556=CARTESIAN_POINT('Ctrl Pts',(1.83272612115297,-0.444293338230862,6.34266823160953));
#4557=CARTESIAN_POINT('Ctrl Pts',(1.64147614223073,-0.592948544581024,6.46460220651928));
#4558=CARTESIAN_POINT('Ctrl Pts',(1.5022165321408,-0.66455929680406,6.55758880230742));
#4559=CARTESIAN_POINT('Ctrl Pts',(1.22448970987637,-0.763214889612529,6.76575702265008));
#4560=CARTESIAN_POINT('Ctrl Pts',(1.08628177383383,-0.79,6.88140722598296));
#4561=CARTESIAN_POINT('Ctrl Pts',(0.96768899981679,-0.79,7.));
#4562=CARTESIAN_POINT('Ctrl Pts',(0.88020875365155,-0.79,7.08748024616524));
#4563=CARTESIAN_POINT('Ctrl Pts',(0.791807275601753,-0.774755581890674,
7.18899251283438));
#4564=CARTESIAN_POINT('Ctrl Pts',(0.683747388356032,-0.714719578864005,
7.34094189934535));
#4565=CARTESIAN_POINT('Ctrl Pts',(0.651565181947462,-0.68858835699378,7.39151504429253));
#4566=CARTESIAN_POINT('Ctrl Pts',(0.596451435323987,-0.624301170571409,
7.487530511074));
#4567=CARTESIAN_POINT('Ctrl Pts',(0.573486312745389,-0.586129881875093,
7.53294329022174));
#4568=CARTESIAN_POINT('Ctrl Pts',(0.539393671847301,-0.508081707721144,
7.60688542088362));
#4569=CARTESIAN_POINT('Ctrl Pts',(0.526116666881167,-0.467880373119377,
7.63868186015549));
#4570=CARTESIAN_POINT('Ctrl Pts',(0.515222755900927,-0.423813975340259,
7.66669461847707));
#4571=CARTESIAN_POINT('',(5.08111831820431,1.95943487863577E-16,3.18162338159264));
#4572=CARTESIAN_POINT('',(0.555634918610405,-1.95943487863577E-16,7.70710678118655));
#4573=CARTESIAN_POINT('Origin',(3.94974746830583,0.,2.05025253169417));
#4574=CARTESIAN_POINT('Origin',(0.5,0.,7.));
#4575=CARTESIAN_POINT('',(0.5,-9.67470971326409E-17,7.79));
#4576=CARTESIAN_POINT('Origin',(0.5,0.,7.));
#4577=CARTESIAN_POINT('Origin',(0.5,0.,7.));
#4578=CARTESIAN_POINT('Origin',(-1.,0.,7.));
#4579=CARTESIAN_POINT('',(-1.62928530890209,-0.477598157450382,6.37071469109791));
#4580=CARTESIAN_POINT('',(-1.62928530890209,0.477598157450382,6.37071469109791));
#4581=CARTESIAN_POINT('Ctrl Pts',(-1.62928530890209,-0.477598157450382,
6.37071469109791));
#4582=CARTESIAN_POINT('Ctrl Pts',(-1.62928530890209,-0.425917629345584,
6.33149158410694));
#4583=CARTESIAN_POINT('Ctrl Pts',(-1.63106209224364,-0.368165804555039,
6.29790350040073));
#4584=CARTESIAN_POINT('Ctrl Pts',(-1.63576347459867,-0.208570757814752,
6.23055387445547));
#4585=CARTESIAN_POINT('Ctrl Pts',(-1.63835569799683,-0.101035232793328,
6.21));
#4586=CARTESIAN_POINT('Ctrl Pts',(-1.63835569799683,0.101035232793328,6.21));
#4587=CARTESIAN_POINT('Ctrl Pts',(-1.63576347459867,0.208570757814752,6.23055387445547));
#4588=CARTESIAN_POINT('Ctrl Pts',(-1.63106209224364,0.368165804555039,6.29790350040073));
#4589=CARTESIAN_POINT('Ctrl Pts',(-1.62928530890209,0.425917629345584,6.33149158410694));
#4590=CARTESIAN_POINT('Ctrl Pts',(-1.62928530890209,0.477598157450382,6.37071469109791));
#4591=CARTESIAN_POINT('',(-0.285822151001587,-1.23689326713883E-16,7.71417784899841));
#4592=CARTESIAN_POINT('Origin',(-1.,0.,7.));
#4593=CARTESIAN_POINT('',(-0.285822151001587,-1.23689326713883E-16,7.71417784899841));
#4594=CARTESIAN_POINT('Origin',(-1.,0.,7.));
#4595=CARTESIAN_POINT('Origin',(-1.,0.,7.));
#4596=CARTESIAN_POINT('',(-1.12609520212919,-0.77987178433381,6.87390479787082));
#4597=CARTESIAN_POINT('Origin',(-1.,0.,7.));
#4598=CARTESIAN_POINT('',(-1.12609520212919,0.77987178433381,6.87390479787082));
#4599=CARTESIAN_POINT('Origin',(-1.,0.,7.));
#4600=CARTESIAN_POINT('Origin',(-1.,0.,7.));
#4601=CARTESIAN_POINT('Origin',(-4.6,0.,7.));
#4602=CARTESIAN_POINT('',(-3.1,9.67470971326409E-17,7.79));
#4603=CARTESIAN_POINT('Origin',(-3.1,0.,7.));
#4604=CARTESIAN_POINT('',(-1.90705627484771,-9.67470971326409E-17,7.79));
#4605=CARTESIAN_POINT('',(-4.6,-9.67470971326409E-17,7.79));
#4606=CARTESIAN_POINT('',(-2.20660681251185,-0.619321665126014,7.49044946233587));
#4607=CARTESIAN_POINT('Origin',(-2.69705627484771,0.,7.));
#4608=CARTESIAN_POINT('Ctrl Pts',(-2.20660681251185,-0.619321665126014,
7.49044946233587));
#4609=CARTESIAN_POINT('Ctrl Pts',(-2.18635739895495,-0.626088765992065,
7.48190421456156));
#4610=CARTESIAN_POINT('Ctrl Pts',(-2.1659929610671,-0.632612788451439,7.47330243874781));
#4611=CARTESIAN_POINT('Ctrl Pts',(-2.00496309821175,-0.682136063507274,
7.40520943133101));
#4612=CARTESIAN_POINT('Ctrl Pts',(-1.86106460441583,-0.713835552448689,
7.34397872871663));
#4613=CARTESIAN_POINT('Ctrl Pts',(-1.61917783401457,-0.754887388656086,
7.23855919060182));
#4614=CARTESIAN_POINT('Ctrl Pts',(-1.48614163670725,-0.771174999515586,
7.18006855577991));
#4615=CARTESIAN_POINT('Ctrl Pts',(-1.34421273277038,-0.782619307675673,
7.10904467456489));
#4616=CARTESIAN_POINT('Ctrl Pts',(-1.30795462851338,-0.78510876895878,7.09020452262876));
#4617=CARTESIAN_POINT('Ctrl Pts',(-1.23823362074948,-0.788767674427645,
7.04876648497192));
#4618=CARTESIAN_POINT('Ctrl Pts',(-1.20466978693098,-0.79,7.02634424192971));
#4619=CARTESIAN_POINT('Ctrl Pts',(-1.17832554500127,-0.79,7.));
#4620=CARTESIAN_POINT('Ctrl Pts',(-1.16484458907882,-0.79,6.98651904407755));
#4621=CARTESIAN_POINT('Ctrl Pts',(-1.15267227667281,-0.789658839214769,
6.97115565787718));
#4622=CARTESIAN_POINT('Ctrl Pts',(-1.13503745407884,-0.787668068667849,
6.93697581829037));
#4623=CARTESIAN_POINT('Ctrl Pts',(-1.12967754955442,-0.785984756040963,
6.91810849353946));
#4624=CARTESIAN_POINT('Ctrl Pts',(-1.12651114233652,-0.782433142969531,
6.89060638382703));
#4625=CARTESIAN_POINT('Ctrl Pts',(-1.12609520212919,-0.781224978053133,
6.88227401083545));
#4626=CARTESIAN_POINT('Ctrl Pts',(-1.12609520212919,-0.77987178433381,6.87390479787082));
#4627=CARTESIAN_POINT('',(-2.20660681251185,0.619321665126014,7.49044946233587));
#4628=CARTESIAN_POINT('Ctrl Pts',(-1.12609520212919,0.77987178433381,6.87390479787082));
#4629=CARTESIAN_POINT('Ctrl Pts',(-1.12609520212919,0.781224978053133,6.88227401083545));
#4630=CARTESIAN_POINT('Ctrl Pts',(-1.12651114233652,0.782433142969531,6.89060638382703));
#4631=CARTESIAN_POINT('Ctrl Pts',(-1.12967754955442,0.785984756040963,6.91810849353946));
#4632=CARTESIAN_POINT('Ctrl Pts',(-1.13503745407884,0.787668068667849,6.93697581829037));
#4633=CARTESIAN_POINT('Ctrl Pts',(-1.15267227667281,0.789658839214769,6.97115565787718));
#4634=CARTESIAN_POINT('Ctrl Pts',(-1.16484458907882,0.79,6.98651904407755));
#4635=CARTESIAN_POINT('Ctrl Pts',(-1.20466978693098,0.79,7.02634424192971));
#4636=CARTESIAN_POINT('Ctrl Pts',(-1.23823362074948,0.788767674427645,7.04876648497192));
#4637=CARTESIAN_POINT('Ctrl Pts',(-1.30795462851338,0.78510876895878,7.09020452262876));
#4638=CARTESIAN_POINT('Ctrl Pts',(-1.34421273277038,0.782619307675673,7.10904467456489));
#4639=CARTESIAN_POINT('Ctrl Pts',(-1.48614163670725,0.771174999515586,7.18006855577991));
#4640=CARTESIAN_POINT('Ctrl Pts',(-1.61917783401457,0.754887388656086,7.23855919060182));
#4641=CARTESIAN_POINT('Ctrl Pts',(-1.86106460441583,0.713835552448689,7.34397872871663));
#4642=CARTESIAN_POINT('Ctrl Pts',(-2.00496309821175,0.682136063507274,7.40520943133101));
#4643=CARTESIAN_POINT('Ctrl Pts',(-2.1659929610671,0.632612788451438,7.47330243874781));
#4644=CARTESIAN_POINT('Ctrl Pts',(-2.18635739895495,0.626088765992065,7.48190421456155));
#4645=CARTESIAN_POINT('Ctrl Pts',(-2.20660681251185,0.619321665126014,7.49044946233587));
#4646=CARTESIAN_POINT('Origin',(-2.69705627484771,0.,7.));
#4647=CARTESIAN_POINT('Origin',(-1.84852813742386,0.,7.84852813742386));
#4648=CARTESIAN_POINT('Origin',(-1.84852813742386,0.,7.84852813742386));
#4649=CARTESIAN_POINT('Origin',(-1.84852813742386,0.,7.84852813742386));
#4650=CARTESIAN_POINT('Origin',(3.1,0.,7.));
#4651=CARTESIAN_POINT('',(3.1,-1.13892152320704E-16,7.93));
#4652=CARTESIAN_POINT('Origin',(3.1,0.,7.));
#4653=CARTESIAN_POINT('',(4.5,1.13892152320704E-16,7.93));
#4654=CARTESIAN_POINT('',(3.1,-1.13892152320704E-16,7.93));
#4655=CARTESIAN_POINT('Origin',(4.5,0.,7.));
#4656=CARTESIAN_POINT('Origin',(3.1,0.,7.));
#4657=CARTESIAN_POINT('',(3.1,-9.67470971326409E-17,7.79));
#4658=CARTESIAN_POINT('Origin',(3.1,0.,7.));
#4659=CARTESIAN_POINT('Origin',(-4.6,0.,7.));
#4660=CARTESIAN_POINT('',(-4.5,-1.13892152320704E-16,7.93));
#4661=CARTESIAN_POINT('Origin',(-4.5,0.,7.));
#4662=CARTESIAN_POINT('',(-3.1,-1.13892152320704E-16,7.93));
#4663=CARTESIAN_POINT('',(-4.6,-1.13892152320704E-16,7.93));
#4664=CARTESIAN_POINT('Origin',(-3.1,0.,7.));
#4665=CARTESIAN_POINT('Origin',(-3.1,0.,7.));
#4666=CARTESIAN_POINT('Origin',(0.5,0.,7.));
#4667=CARTESIAN_POINT('',(0.5,-9.67470971326409E-17,7.79));
#4668=CARTESIAN_POINT('Origin',(3.3840620433566,0.,2.61593795664341));
#4669=CARTESIAN_POINT('',(5.50538238691624,-3.67394039744206E-16,4.73725830020305));
#4670=CARTESIAN_POINT('Origin',(3.3840620433566,0.,2.61593795664341));
#4671=CARTESIAN_POINT('',(4.79827560572969,2.44929359829471E-16,4.0301515190165));
#4672=CARTESIAN_POINT('Origin',(3.3840620433566,0.,2.61593795664341));
#4673=CARTESIAN_POINT('Origin',(3.3840620433566,0.,2.61593795664341));
#4674=CARTESIAN_POINT('',(6.07106781186548,-3.67394039744206E-16,4.17157287525381));
#4675=CARTESIAN_POINT('Origin',(3.94974746830583,0.,2.05025253169417));
#4676=CARTESIAN_POINT('',(5.50538238691624,-3.67394039744206E-16,4.73725830020305));
#4677=CARTESIAN_POINT('Origin',(-1.,0.,7.));
#4678=CARTESIAN_POINT('',(3.82842712474619,-2.44929359829471E-16,5.));
#4679=CARTESIAN_POINT('',(0.414213562373095,-2.44929359829471E-16,8.4142135623731));
#4680=CARTESIAN_POINT('',(-1.,-2.,7.));
#4681=CARTESIAN_POINT('Origin',(-1.,0.,7.));
#4682=CARTESIAN_POINT('',(-1.,2.,7.));
#4683=CARTESIAN_POINT('Origin',(-1.,0.,7.));
#4684=CARTESIAN_POINT('Origin',(-1.,0.,7.));
#4685=CARTESIAN_POINT('Origin',(3.94974746830583,0.,2.05025253169417));
#4686=CARTESIAN_POINT('Origin',(-4.5,0.,7.));
#4687=CARTESIAN_POINT('',(4.5,-2.44929359829471E-16,9.));
#4688=CARTESIAN_POINT('Origin',(4.5,0.,7.));
#4689=CARTESIAN_POINT('',(-4.5,-2.44929359829471E-16,9.));
#4690=CARTESIAN_POINT('',(-4.5,-2.44929359829471E-16,9.));
#4691=CARTESIAN_POINT('Origin',(-4.5,0.,7.));
#4692=CARTESIAN_POINT('Origin',(4.5,0.,7.));
#4693=CARTESIAN_POINT('Origin',(-4.5,0.,7.));
#8843=UNCERTAINTY_MEASURE_WITH_UNIT(LENGTH_MEASURE(0.001),#8865,
'DISTANCE_ACCURACY_VALUE',
'Maximum model space distance between geometric entities at asserted c
onnectivities');
#8852=UNCERTAINTY_MEASURE_WITH_UNIT(LENGTH_MEASURE(0.001),#8865,
'DISTANCE_ACCURACY_VALUE',
'Maximum model space distance between geometric entities at asserted c
onnectivities');
#8855=(
GEOMETRIC_REPRESENTATION_CONTEXT(3)
GLOBAL_UNCERTAINTY_ASSIGNED_CONTEXT((#8843))
GLOBAL_UNIT_ASSIGNED_CONTEXT((#8865,#8867,#8868))
REPRESENTATION_CONTEXT('','3D')
);
#8864=(
GEOMETRIC_REPRESENTATION_CONTEXT(3)
GLOBAL_UNCERTAINTY_ASSIGNED_CONTEXT((#8852))
GLOBAL_UNIT_ASSIGNED_CONTEXT((#8865,#8867,#8868))
REPRESENTATION_CONTEXT('','3D')
);
#8865=(
LENGTH_UNIT()
NAMED_UNIT(*)
SI_UNIT(.CENTI.,.METRE.)
);
#8867=(
NAMED_UNIT(*)
PLANE_ANGLE_UNIT()
SI_UNIT($,.RADIAN.)
);
#8868=(
NAMED_UNIT(*)
SI_UNIT($,.STERADIAN.)
SOLID_ANGLE_UNIT()
);
#8871=SHAPE_DEFINITION_REPRESENTATION(#8882,#8907);
#8882=PRODUCT_DEFINITION_SHAPE('',$,#8919);
#8907=SHAPE_REPRESENTATION('',(#3495),#8855);
#8916=PRODUCT_DEFINITION_CONTEXT('part definition',#8951,'design');
#8919=PRODUCT_DEFINITION('Round-chamber strainer housing',
'Round-chamber strainer housing',#8930,#8916);
#8930=PRODUCT_DEFINITION_FORMATION('',$,#8955);
#8951=APPLICATION_CONTEXT(
'Core Data for Automotive Mechanical Design Process');
#8952=PRODUCT_CONTEXT('part definition',#8951,'mechanical');
#8955=PRODUCT('Round-chamber strainer housing',
'Round-chamber strainer housing','Round-chamber strainer housing',(#8952));
#9006=COLOUR_RGB('Dark Blue',0.08,0.2,0.34);
#9007=FILL_AREA_STYLE_COLOUR('',#9006);
#9008=FILL_AREA_STYLE('',(#9007));
#9009=SURFACE_STYLE_FILL_AREA(#9008);
#9010=SURFACE_SIDE_STYLE('',(#9009));
#9011=SURFACE_STYLE_USAGE(.BOTH.,#9010);
#9012=PRESENTATION_STYLE_ASSIGNMENT((#9011));
ENDSEC;
END-ISO-10303-21;
